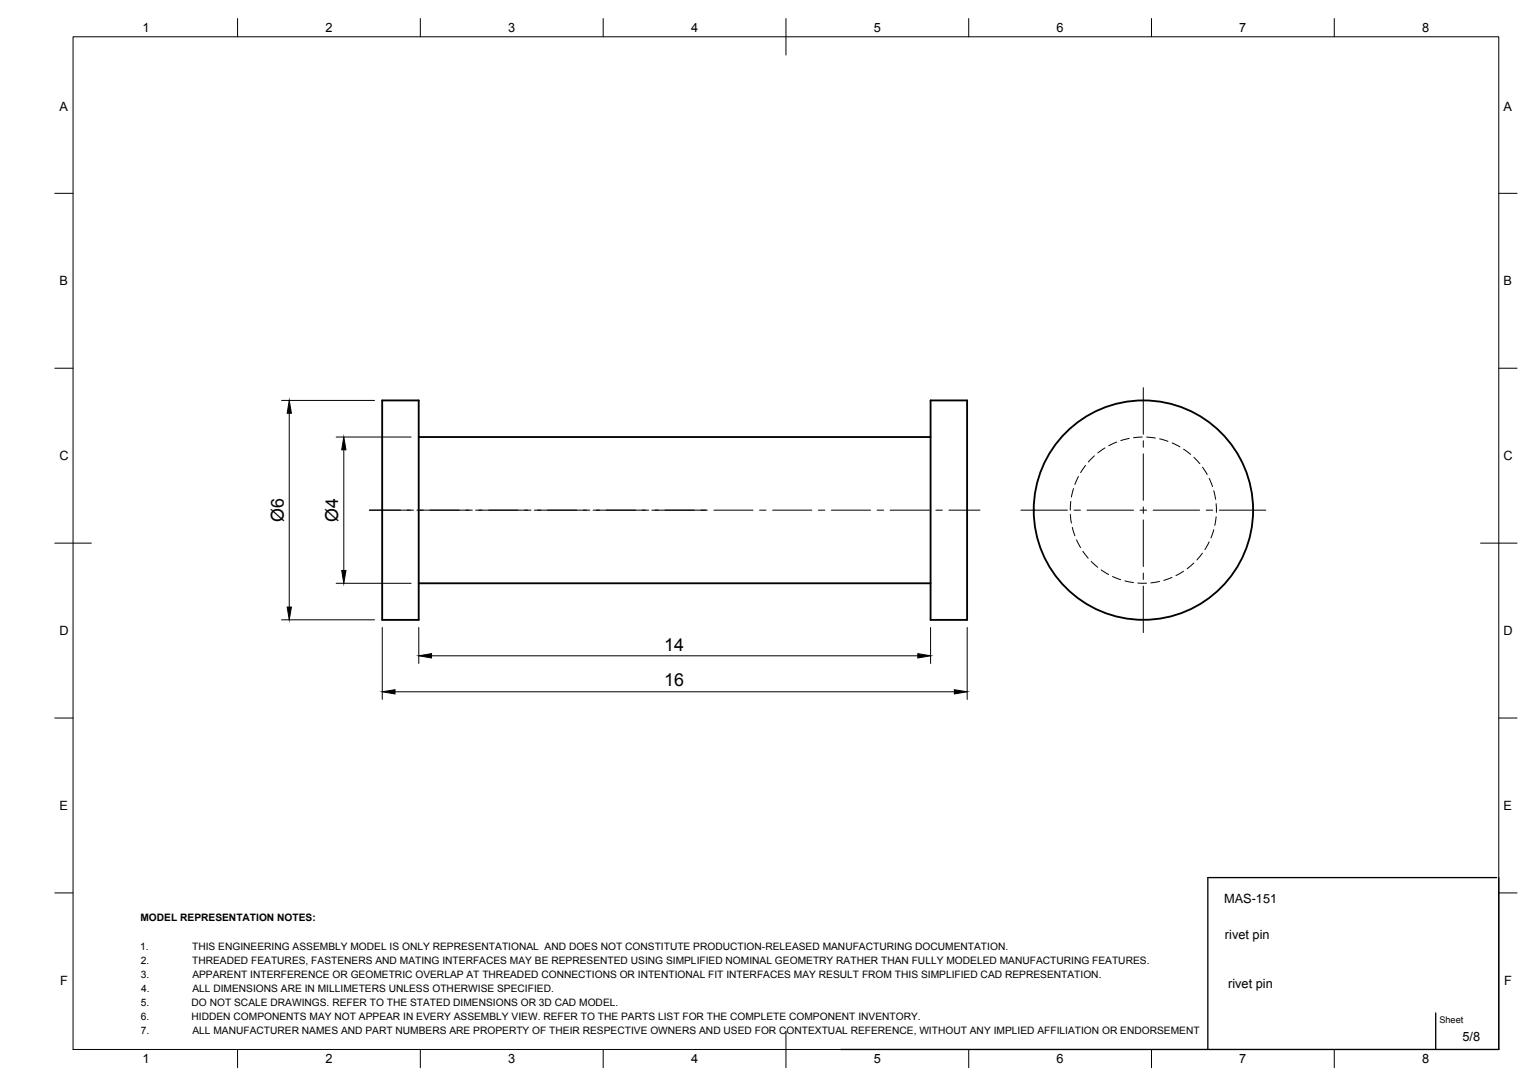
ISO-10303-21;
HEADER;
/* Generated by software containing ST-Developer
 * from STEP Tools, Inc. (www.steptools.com) 
 */

FILE_DESCRIPTION(
/* description */ ('STEP AP214'),
/* implementation_level */ '2;1');

FILE_NAME(
/* name */ 'rivet pin.step',
/* time_stamp */ '2026-11-04T19:14:12-08:00',
/* author */ (''),
/* organization */ (''),
/* preprocessor_version */ 'ST-DEVELOPER v20.2',
/* originating_system */ 'Autodesk Translation Framework v15.17.0.0',
/* authorisation */ '');

FILE_SCHEMA (('AUTOMOTIVE_DESIGN { 1 0 10303 214 3 1 1 }'));
ENDSEC;

DATA;
#10=MECHANICAL_DESIGN_GEOMETRIC_PRESENTATION_REPRESENTATION('',(#105),#5990);
#91=SHAPE_REPRESENTATION_RELATIONSHIP('SRR','None',#6027,#98);
#98=ADVANCED_BREP_SHAPE_REPRESENTATION('',(#112),#5989);
#105=STYLED_ITEM('',(#6069),#112);
#112=MANIFOLD_SOLID_BREP('Body1',#3275);
#135=FACE_BOUND('',#618,.T.);
#136=FACE_BOUND('',#621,.T.);
#238=PLANE('',#3672);
#239=PLANE('',#3673);
#240=PLANE('',#3674);
#241=PLANE('',#3675);
#413=FACE_OUTER_BOUND('',#613,.T.);
#414=FACE_OUTER_BOUND('',#614,.T.);
#415=FACE_OUTER_BOUND('',#615,.T.);
#416=FACE_OUTER_BOUND('',#616,.T.);
#417=FACE_OUTER_BOUND('',#617,.T.);
#418=FACE_OUTER_BOUND('',#619,.T.);
#419=FACE_OUTER_BOUND('',#620,.T.);
#613=EDGE_LOOP('',(#3010,#3011,#3012,#3013));
#614=EDGE_LOOP('',(#3014,#3015,#3016,#3017));
#615=EDGE_LOOP('',(#3018,#3019,#3020,#3021));
#616=EDGE_LOOP('',(#3022));
#617=EDGE_LOOP('',(#3023));
#618=EDGE_LOOP('',(#3024));
#619=EDGE_LOOP('',(#3025));
#620=EDGE_LOOP('',(#3026));
#621=EDGE_LOOP('',(#3027));
#922=LINE('',#5946,#1225);
#923=LINE('',#5952,#1226);
#924=LINE('',#5958,#1227);
#1225=VECTOR('',#4607,3.);
#1226=VECTOR('',#4614,3.);
#1227=VECTOR('',#4621,2.);
#1350=CIRCLE('',#3664,3.);
#1351=CIRCLE('',#3665,3.);
#1352=CIRCLE('',#3667,3.);
#1353=CIRCLE('',#3668,3.);
#1354=CIRCLE('',#3670,2.);
#1355=CIRCLE('',#3671,2.);
#1645=VERTEX_POINT('',#5943);
#1646=VERTEX_POINT('',#5945);
#1647=VERTEX_POINT('',#5949);
#1648=VERTEX_POINT('',#5951);
#1649=VERTEX_POINT('',#5955);
#1650=VERTEX_POINT('',#5957);
#2101=EDGE_CURVE('',#1645,#1645,#1350,.T.);
#2102=EDGE_CURVE('',#1645,#1646,#922,.T.);
#2103=EDGE_CURVE('',#1646,#1646,#1351,.T.);
#2104=EDGE_CURVE('',#1647,#1647,#1352,.T.);
#2105=EDGE_CURVE('',#1647,#1648,#923,.T.);
#2106=EDGE_CURVE('',#1648,#1648,#1353,.T.);
#2107=EDGE_CURVE('',#1649,#1649,#1354,.T.);
#2108=EDGE_CURVE('',#1649,#1650,#924,.T.);
#2109=EDGE_CURVE('',#1650,#1650,#1355,.T.);
#3010=ORIENTED_EDGE('',*,*,#2101,.F.);
#3011=ORIENTED_EDGE('',*,*,#2102,.T.);
#3012=ORIENTED_EDGE('',*,*,#2103,.T.);
#3013=ORIENTED_EDGE('',*,*,#2102,.F.);
#3014=ORIENTED_EDGE('',*,*,#2104,.T.);
#3015=ORIENTED_EDGE('',*,*,#2105,.T.);
#3016=ORIENTED_EDGE('',*,*,#2106,.F.);
#3017=ORIENTED_EDGE('',*,*,#2105,.F.);
#3018=ORIENTED_EDGE('',*,*,#2107,.T.);
#3019=ORIENTED_EDGE('',*,*,#2108,.T.);
#3020=ORIENTED_EDGE('',*,*,#2109,.F.);
#3021=ORIENTED_EDGE('',*,*,#2108,.F.);
#3022=ORIENTED_EDGE('',*,*,#2106,.T.);
#3023=ORIENTED_EDGE('',*,*,#2104,.F.);
#3024=ORIENTED_EDGE('',*,*,#2109,.T.);
#3025=ORIENTED_EDGE('',*,*,#2103,.F.);
#3026=ORIENTED_EDGE('',*,*,#2101,.T.);
#3027=ORIENTED_EDGE('',*,*,#2107,.F.);
#3088=CYLINDRICAL_SURFACE('',#3663,3.);
#3089=CYLINDRICAL_SURFACE('',#3666,3.);
#3090=CYLINDRICAL_SURFACE('',#3669,2.);
#3262=ADVANCED_FACE('',(#413),#3088,.T.);
#3263=ADVANCED_FACE('',(#414),#3089,.T.);
#3264=ADVANCED_FACE('',(#415),#3090,.T.);
#3265=ADVANCED_FACE('',(#416),#238,.T.);
#3266=ADVANCED_FACE('',(#417,#135),#239,.F.);
#3267=ADVANCED_FACE('',(#418),#240,.T.);
#3268=ADVANCED_FACE('',(#419,#136),#241,.F.);
#3275=CLOSED_SHELL('',(#3262,#3263,#3264,#3265,#3266,#3267,#3268));
#3662=AXIS2_PLACEMENT_3D('',#5941,#4601,#4602);
#3663=AXIS2_PLACEMENT_3D('',#5942,#4603,#4604);
#3664=AXIS2_PLACEMENT_3D('',#5944,#4605,#4606);
#3665=AXIS2_PLACEMENT_3D('',#5947,#4608,#4609);
#3666=AXIS2_PLACEMENT_3D('',#5948,#4610,#4611);
#3667=AXIS2_PLACEMENT_3D('',#5950,#4612,#4613);
#3668=AXIS2_PLACEMENT_3D('',#5953,#4615,#4616);
#3669=AXIS2_PLACEMENT_3D('',#5954,#4617,#4618);
#3670=AXIS2_PLACEMENT_3D('',#5956,#4619,#4620);
#3671=AXIS2_PLACEMENT_3D('',#5959,#4622,#4623);
#3672=AXIS2_PLACEMENT_3D('',#5960,#4624,#4625);
#3673=AXIS2_PLACEMENT_3D('',#5961,#4626,#4627);
#3674=AXIS2_PLACEMENT_3D('',#5962,#4628,#4629);
#3675=AXIS2_PLACEMENT_3D('',#5963,#4630,#4631);
#4601=DIRECTION('axis',(0.,0.,1.));
#4602=DIRECTION('refdir',(1.,0.,0.));
#4603=DIRECTION('center_axis',(0.,0.,1.));
#4604=DIRECTION('ref_axis',(-1.,0.,0.));
#4605=DIRECTION('center_axis',(0.,0.,1.));
#4606=DIRECTION('ref_axis',(1.,0.,0.));
#4607=DIRECTION('',(0.,0.,-1.));
#4608=DIRECTION('center_axis',(0.,0.,1.));
#4609=DIRECTION('ref_axis',(1.,0.,0.));
#4610=DIRECTION('center_axis',(0.,0.,-1.));
#4611=DIRECTION('ref_axis',(-1.,0.,0.));
#4612=DIRECTION('center_axis',(0.,0.,1.));
#4613=DIRECTION('ref_axis',(1.,0.,0.));
#4614=DIRECTION('',(0.,0.,1.));
#4615=DIRECTION('center_axis',(0.,0.,1.));
#4616=DIRECTION('ref_axis',(1.,0.,0.));
#4617=DIRECTION('center_axis',(0.,0.,-1.));
#4618=DIRECTION('ref_axis',(-1.,0.,0.));
#4619=DIRECTION('center_axis',(0.,0.,1.));
#4620=DIRECTION('ref_axis',(1.,0.,0.));
#4621=DIRECTION('',(0.,0.,1.));
#4622=DIRECTION('center_axis',(0.,0.,1.));
#4623=DIRECTION('ref_axis',(1.,0.,0.));
#4624=DIRECTION('center_axis',(0.,0.,1.));
#4625=DIRECTION('ref_axis',(1.,0.,0.));
#4626=DIRECTION('center_axis',(0.,0.,1.));
#4627=DIRECTION('ref_axis',(1.,0.,0.));
#4628=DIRECTION('center_axis',(0.,0.,-1.));
#4629=DIRECTION('ref_axis',(1.,0.,0.));
#4630=DIRECTION('center_axis',(0.,0.,-1.));
#4631=DIRECTION('ref_axis',(1.,0.,0.));
#5941=CARTESIAN_POINT('',(0.,0.,0.));
#5942=CARTESIAN_POINT('Origin',(5.,-15.2931109241333,-8.));
#5943=CARTESIAN_POINT('',(8.,-15.2931109241333,-7.));
#5944=CARTESIAN_POINT('Origin',(5.,-15.2931109241333,-7.));
#5945=CARTESIAN_POINT('',(8.,-15.2931109241333,-8.));
#5946=CARTESIAN_POINT('',(8.,-15.2931109241333,-8.));
#5947=CARTESIAN_POINT('Origin',(5.,-15.2931109241333,-8.));
#5948=CARTESIAN_POINT('Origin',(5.,-15.2931109241333,8.));
#5949=CARTESIAN_POINT('',(8.,-15.2931109241333,7.));
#5950=CARTESIAN_POINT('Origin',(5.,-15.2931109241333,7.));
#5951=CARTESIAN_POINT('',(8.,-15.2931109241333,8.));
#5952=CARTESIAN_POINT('',(8.,-15.2931109241333,8.));
#5953=CARTESIAN_POINT('Origin',(5.,-15.2931109241333,8.));
#5954=CARTESIAN_POINT('Origin',(5.,-15.2931109241333,7.));
#5955=CARTESIAN_POINT('',(7.,-15.2931109241333,-7.));
#5956=CARTESIAN_POINT('Origin',(5.,-15.2931109241333,-7.));
#5957=CARTESIAN_POINT('',(7.,-15.2931109241333,7.));
#5958=CARTESIAN_POINT('',(7.,-15.2931109241333,7.));
#5959=CARTESIAN_POINT('Origin',(5.,-15.2931109241333,7.));
#5960=CARTESIAN_POINT('Origin',(5.,-15.2931109241333,8.));
#5961=CARTESIAN_POINT('Origin',(5.,-15.2931109241333,7.));
#5962=CARTESIAN_POINT('Origin',(5.,-15.2931109241333,-8.));
#5963=CARTESIAN_POINT('Origin',(5.,-15.2931109241333,-7.));
#5980=UNCERTAINTY_MEASURE_WITH_UNIT(LENGTH_MEASURE(0.01),#5991,
'DISTANCE_ACCURACY_VALUE',
'Maximum model space distance between geometric entities at asserted c
onnectivities');
#5981=UNCERTAINTY_MEASURE_WITH_UNIT(LENGTH_MEASURE(0.01),#5991,
'DISTANCE_ACCURACY_VALUE',
'Maximum model space distance between geometric entities at asserted c
onnectivities');
#5989=(
GEOMETRIC_REPRESENTATION_CONTEXT(3)
GLOBAL_UNCERTAINTY_ASSIGNED_CONTEXT((#5980))
GLOBAL_UNIT_ASSIGNED_CONTEXT((#5991,#5993,#5994))
REPRESENTATION_CONTEXT('','3D')
);
#5990=(
GEOMETRIC_REPRESENTATION_CONTEXT(3)
GLOBAL_UNCERTAINTY_ASSIGNED_CONTEXT((#5981))
GLOBAL_UNIT_ASSIGNED_CONTEXT((#5991,#5993,#5994))
REPRESENTATION_CONTEXT('','3D')
);
#5991=(
LENGTH_UNIT()
NAMED_UNIT(*)
SI_UNIT(.MILLI.,.METRE.)
);
#5993=(
NAMED_UNIT(*)
PLANE_ANGLE_UNIT()
SI_UNIT($,.RADIAN.)
);
#5994=(
NAMED_UNIT(*)
SI_UNIT($,.STERADIAN.)
SOLID_ANGLE_UNIT()
);
#6002=SHAPE_DEFINITION_REPRESENTATION(#6010,#6027);
#6010=PRODUCT_DEFINITION_SHAPE('',$,#6036);
#6027=SHAPE_REPRESENTATION('',(#3662),#5989);
#6028=PRODUCT_DEFINITION_CONTEXT('part definition',#6054,'design');
#6036=PRODUCT_DEFINITION('rivet pin','rivet pin',#6044,#6028);
#6044=PRODUCT_DEFINITION_FORMATION('',$,#6063);
#6054=APPLICATION_CONTEXT(
'Core Data for Automotive Mechanical Design Process');
#6055=PRODUCT_CONTEXT('part definition',#6054,'mechanical');
#6063=PRODUCT('rivet pin','rivet pin',$,(#6055));
#6069=PRESENTATION_STYLE_ASSIGNMENT((#6075));
#6075=SURFACE_STYLE_USAGE(.BOTH.,#6081);
#6081=SURFACE_SIDE_STYLE('',(#6087));
#6087=SURFACE_STYLE_FILL_AREA(#6093);
#6093=FILL_AREA_STYLE('Opaque(122,133,145)',(#6099));
#6099=FILL_AREA_STYLE_COLOUR('Opaque(122,133,145)',#6105);
#6105=COLOUR_RGB('Opaque(122,133,145)',0.47843137254902,0.52156862745098,
0.568627450980392);
ENDSEC;
END-ISO-10303-21;
